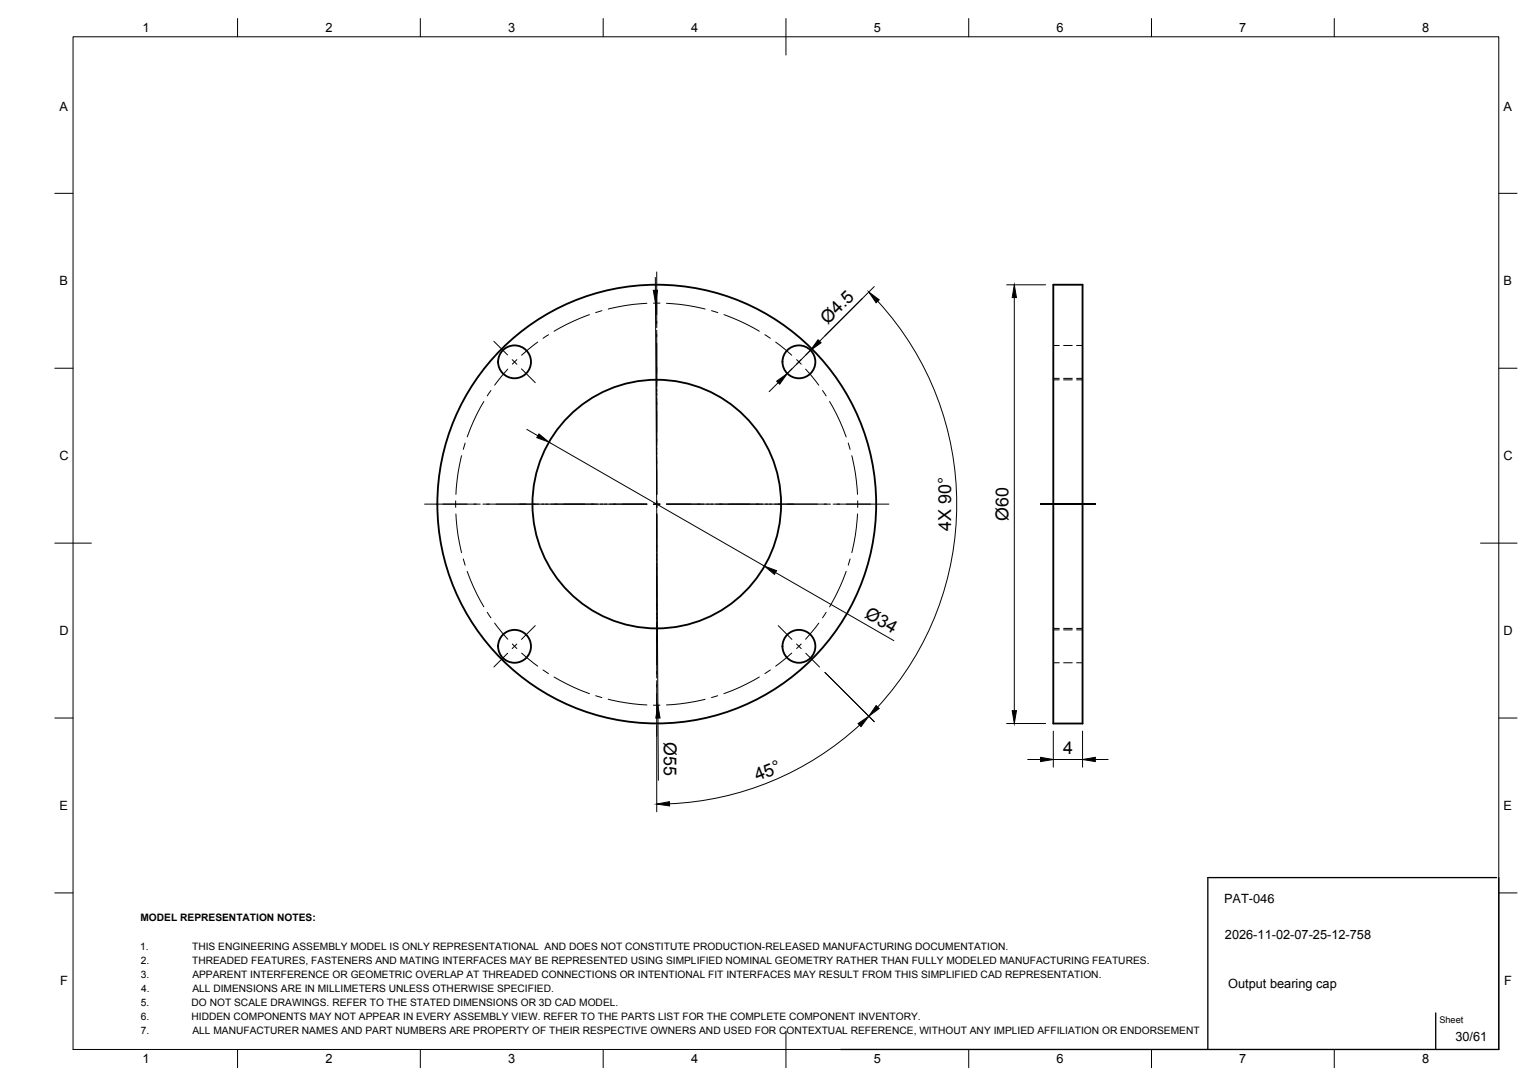
ISO-10303-21;
HEADER;
/* Generated by software containing ST-Developer
 * from STEP Tools, Inc. (www.steptools.com) 
 */

FILE_DESCRIPTION(
/* description */ ('Gear mesh backlash fixture'),
/* implementation_level */ '2;1');

FILE_NAME(
/* name */ 'Output bearing cap.step',
/* time_stamp */ '2026-10-28T03:26:00-07:00',
/* author */ (''),
/* organization */ (''),
/* preprocessor_version */ 'ST-DEVELOPER v20.2',
/* originating_system */ 'Autodesk Translation Framework v15.17.0.0',
/* authorisation */ '');

FILE_SCHEMA (('AUTOMOTIVE_DESIGN { 1 0 10303 214 3 1 1 }'));
ENDSEC;

DATA;
#10=MECHANICAL_DESIGN_GEOMETRIC_PRESENTATION_REPRESENTATION('',(#1045),#57900);
#938=SHAPE_REPRESENTATION_RELATIONSHIP('SRR','None',#58135,#988);
#988=ADVANCED_BREP_SHAPE_REPRESENTATION('',(#1109),#57868);
#1045=STYLED_ITEM('',(#58465),#1109);
#1109=MANIFOLD_SOLID_BREP('Body1',#13606);
#1266=FACE_BOUND('',#2861,.T.);
#1267=FACE_BOUND('',#2862,.T.);
#1268=FACE_BOUND('',#2863,.T.);
#1269=FACE_BOUND('',#2864,.T.);
#1270=FACE_BOUND('',#2865,.T.);
#1271=FACE_BOUND('',#2867,.T.);
#1272=FACE_BOUND('',#2868,.T.);
#1273=FACE_BOUND('',#2869,.T.);
#1274=FACE_BOUND('',#2870,.T.);
#1275=FACE_BOUND('',#2871,.T.);
#1472=PLANE('',#14799);
#1473=PLANE('',#14800);
#1966=FACE_OUTER_BOUND('',#2854,.T.);
#1967=FACE_OUTER_BOUND('',#2855,.T.);
#1968=FACE_OUTER_BOUND('',#2856,.T.);
#1969=FACE_OUTER_BOUND('',#2857,.T.);
#1970=FACE_OUTER_BOUND('',#2858,.T.);
#1971=FACE_OUTER_BOUND('',#2859,.T.);
#1972=FACE_OUTER_BOUND('',#2860,.T.);
#1973=FACE_OUTER_BOUND('',#2866,.T.);
#2854=EDGE_LOOP('',(#10089,#10090,#10091,#10092));
#2855=EDGE_LOOP('',(#10093,#10094,#10095,#10096));
#2856=EDGE_LOOP('',(#10097,#10098,#10099,#10100));
#2857=EDGE_LOOP('',(#10101,#10102,#10103,#10104));
#2858=EDGE_LOOP('',(#10105,#10106,#10107,#10108));
#2859=EDGE_LOOP('',(#10109,#10110,#10111,#10112));
#2860=EDGE_LOOP('',(#10113));
#2861=EDGE_LOOP('',(#10114));
#2862=EDGE_LOOP('',(#10115));
#2863=EDGE_LOOP('',(#10116));
#2864=EDGE_LOOP('',(#10117));
#2865=EDGE_LOOP('',(#10118));
#2866=EDGE_LOOP('',(#10119));
#2867=EDGE_LOOP('',(#10120));
#2868=EDGE_LOOP('',(#10121));
#2869=EDGE_LOOP('',(#10122));
#2870=EDGE_LOOP('',(#10123));
#2871=EDGE_LOOP('',(#10124));
#3709=LINE('',#21009,#4598);
#3710=LINE('',#21015,#4599);
#3711=LINE('',#21021,#4600);
#3712=LINE('',#21027,#4601);
#3713=LINE('',#21033,#4602);
#3714=LINE('',#21039,#4603);
#4598=VECTOR('',#17052,0.225);
#4599=VECTOR('',#17059,0.225);
#4600=VECTOR('',#17066,0.225);
#4601=VECTOR('',#17073,0.225000000000001);
#4602=VECTOR('',#17080,1.7);
#4603=VECTOR('',#17087,3.);
#5471=CIRCLE('',#14782,0.225);
#5472=CIRCLE('',#14783,0.225);
#5473=CIRCLE('',#14785,0.225);
#5474=CIRCLE('',#14786,0.225);
#5475=CIRCLE('',#14788,0.225);
#5476=CIRCLE('',#14789,0.225);
#5477=CIRCLE('',#14791,0.225000000000001);
#5478=CIRCLE('',#14792,0.225000000000001);
#5479=CIRCLE('',#14794,1.7);
#5480=CIRCLE('',#14795,1.7);
#5481=CIRCLE('',#14797,3.);
#5482=CIRCLE('',#14798,3.);
#6187=VERTEX_POINT('',#21006);
#6188=VERTEX_POINT('',#21008);
#6189=VERTEX_POINT('',#21012);
#6190=VERTEX_POINT('',#21014);
#6191=VERTEX_POINT('',#21018);
#6192=VERTEX_POINT('',#21020);
#6193=VERTEX_POINT('',#21024);
#6194=VERTEX_POINT('',#21026);
#6195=VERTEX_POINT('',#21030);
#6196=VERTEX_POINT('',#21032);
#6197=VERTEX_POINT('',#21036);
#6198=VERTEX_POINT('',#21038);
#7631=EDGE_CURVE('',#6187,#6187,#5471,.T.);
#7632=EDGE_CURVE('',#6187,#6188,#3709,.T.);
#7633=EDGE_CURVE('',#6188,#6188,#5472,.T.);
#7634=EDGE_CURVE('',#6189,#6189,#5473,.T.);
#7635=EDGE_CURVE('',#6189,#6190,#3710,.T.);
#7636=EDGE_CURVE('',#6190,#6190,#5474,.T.);
#7637=EDGE_CURVE('',#6191,#6191,#5475,.T.);
#7638=EDGE_CURVE('',#6191,#6192,#3711,.T.);
#7639=EDGE_CURVE('',#6192,#6192,#5476,.T.);
#7640=EDGE_CURVE('',#6193,#6193,#5477,.T.);
#7641=EDGE_CURVE('',#6193,#6194,#3712,.T.);
#7642=EDGE_CURVE('',#6194,#6194,#5478,.T.);
#7643=EDGE_CURVE('',#6195,#6195,#5479,.T.);
#7644=EDGE_CURVE('',#6195,#6196,#3713,.T.);
#7645=EDGE_CURVE('',#6196,#6196,#5480,.T.);
#7646=EDGE_CURVE('',#6197,#6197,#5481,.T.);
#7647=EDGE_CURVE('',#6197,#6198,#3714,.T.);
#7648=EDGE_CURVE('',#6198,#6198,#5482,.T.);
#10089=ORIENTED_EDGE('',*,*,#7631,.F.);
#10090=ORIENTED_EDGE('',*,*,#7632,.T.);
#10091=ORIENTED_EDGE('',*,*,#7633,.F.);
#10092=ORIENTED_EDGE('',*,*,#7632,.F.);
#10093=ORIENTED_EDGE('',*,*,#7634,.F.);
#10094=ORIENTED_EDGE('',*,*,#7635,.T.);
#10095=ORIENTED_EDGE('',*,*,#7636,.F.);
#10096=ORIENTED_EDGE('',*,*,#7635,.F.);
#10097=ORIENTED_EDGE('',*,*,#7637,.F.);
#10098=ORIENTED_EDGE('',*,*,#7638,.T.);
#10099=ORIENTED_EDGE('',*,*,#7639,.F.);
#10100=ORIENTED_EDGE('',*,*,#7638,.F.);
#10101=ORIENTED_EDGE('',*,*,#7640,.F.);
#10102=ORIENTED_EDGE('',*,*,#7641,.T.);
#10103=ORIENTED_EDGE('',*,*,#7642,.F.);
#10104=ORIENTED_EDGE('',*,*,#7641,.F.);
#10105=ORIENTED_EDGE('',*,*,#7643,.F.);
#10106=ORIENTED_EDGE('',*,*,#7644,.T.);
#10107=ORIENTED_EDGE('',*,*,#7645,.T.);
#10108=ORIENTED_EDGE('',*,*,#7644,.F.);
#10109=ORIENTED_EDGE('',*,*,#7646,.F.);
#10110=ORIENTED_EDGE('',*,*,#7647,.T.);
#10111=ORIENTED_EDGE('',*,*,#7648,.T.);
#10112=ORIENTED_EDGE('',*,*,#7647,.F.);
#10113=ORIENTED_EDGE('',*,*,#7646,.T.);
#10114=ORIENTED_EDGE('',*,*,#7643,.T.);
#10115=ORIENTED_EDGE('',*,*,#7642,.T.);
#10116=ORIENTED_EDGE('',*,*,#7639,.T.);
#10117=ORIENTED_EDGE('',*,*,#7636,.T.);
#10118=ORIENTED_EDGE('',*,*,#7633,.T.);
#10119=ORIENTED_EDGE('',*,*,#7648,.F.);
#10120=ORIENTED_EDGE('',*,*,#7645,.F.);
#10121=ORIENTED_EDGE('',*,*,#7640,.T.);
#10122=ORIENTED_EDGE('',*,*,#7637,.T.);
#10123=ORIENTED_EDGE('',*,*,#7634,.T.);
#10124=ORIENTED_EDGE('',*,*,#7631,.T.);
#12691=CYLINDRICAL_SURFACE('',#14781,0.225);
#12692=CYLINDRICAL_SURFACE('',#14784,0.225);
#12693=CYLINDRICAL_SURFACE('',#14787,0.225);
#12694=CYLINDRICAL_SURFACE('',#14790,0.225000000000001);
#12695=CYLINDRICAL_SURFACE('',#14793,1.7);
#12696=CYLINDRICAL_SURFACE('',#14796,3.);
#13083=ADVANCED_FACE('',(#1966),#12691,.F.);
#13084=ADVANCED_FACE('',(#1967),#12692,.F.);
#13085=ADVANCED_FACE('',(#1968),#12693,.F.);
#13086=ADVANCED_FACE('',(#1969),#12694,.F.);
#13087=ADVANCED_FACE('',(#1970),#12695,.F.);
#13088=ADVANCED_FACE('',(#1971),#12696,.T.);
#13089=ADVANCED_FACE('',(#1972,#1266,#1267,#1268,#1269,#1270),#1472,.T.);
#13090=ADVANCED_FACE('',(#1973,#1271,#1272,#1273,#1274,#1275),#1473,.F.);
#13606=CLOSED_SHELL('',(#13083,#13084,#13085,#13086,#13087,#13088,#13089,
#13090));
#14780=AXIS2_PLACEMENT_3D('',#21004,#17046,#17047);
#14781=AXIS2_PLACEMENT_3D('',#21005,#17048,#17049);
#14782=AXIS2_PLACEMENT_3D('',#21007,#17050,#17051);
#14783=AXIS2_PLACEMENT_3D('',#21010,#17053,#17054);
#14784=AXIS2_PLACEMENT_3D('',#21011,#17055,#17056);
#14785=AXIS2_PLACEMENT_3D('',#21013,#17057,#17058);
#14786=AXIS2_PLACEMENT_3D('',#21016,#17060,#17061);
#14787=AXIS2_PLACEMENT_3D('',#21017,#17062,#17063);
#14788=AXIS2_PLACEMENT_3D('',#21019,#17064,#17065);
#14789=AXIS2_PLACEMENT_3D('',#21022,#17067,#17068);
#14790=AXIS2_PLACEMENT_3D('',#21023,#17069,#17070);
#14791=AXIS2_PLACEMENT_3D('',#21025,#17071,#17072);
#14792=AXIS2_PLACEMENT_3D('',#21028,#17074,#17075);
#14793=AXIS2_PLACEMENT_3D('',#21029,#17076,#17077);
#14794=AXIS2_PLACEMENT_3D('',#21031,#17078,#17079);
#14795=AXIS2_PLACEMENT_3D('',#21034,#17081,#17082);
#14796=AXIS2_PLACEMENT_3D('',#21035,#17083,#17084);
#14797=AXIS2_PLACEMENT_3D('',#21037,#17085,#17086);
#14798=AXIS2_PLACEMENT_3D('',#21040,#17088,#17089);
#14799=AXIS2_PLACEMENT_3D('',#21041,#17090,#17091);
#14800=AXIS2_PLACEMENT_3D('',#21042,#17092,#17093);
#17046=DIRECTION('axis',(0.,0.,1.));
#17047=DIRECTION('refdir',(1.,0.,0.));
#17048=DIRECTION('center_axis',(0.,0.,1.));
#17049=DIRECTION('ref_axis',(1.,0.,0.));
#17050=DIRECTION('center_axis',(0.,0.,1.));
#17051=DIRECTION('ref_axis',(1.,0.,0.));
#17052=DIRECTION('',(0.,0.,1.));
#17053=DIRECTION('center_axis',(0.,0.,-1.));
#17054=DIRECTION('ref_axis',(1.,0.,0.));
#17055=DIRECTION('center_axis',(0.,0.,1.));
#17056=DIRECTION('ref_axis',(1.,0.,0.));
#17057=DIRECTION('center_axis',(0.,0.,1.));
#17058=DIRECTION('ref_axis',(1.,0.,0.));
#17059=DIRECTION('',(0.,0.,1.));
#17060=DIRECTION('center_axis',(0.,0.,-1.));
#17061=DIRECTION('ref_axis',(1.,0.,0.));
#17062=DIRECTION('center_axis',(0.,0.,1.));
#17063=DIRECTION('ref_axis',(1.,0.,0.));
#17064=DIRECTION('center_axis',(0.,0.,1.));
#17065=DIRECTION('ref_axis',(1.,0.,0.));
#17066=DIRECTION('',(0.,0.,1.));
#17067=DIRECTION('center_axis',(0.,0.,-1.));
#17068=DIRECTION('ref_axis',(1.,0.,0.));
#17069=DIRECTION('center_axis',(0.,0.,1.));
#17070=DIRECTION('ref_axis',(1.,0.,0.));
#17071=DIRECTION('center_axis',(0.,0.,1.));
#17072=DIRECTION('ref_axis',(1.,0.,0.));
#17073=DIRECTION('',(0.,0.,1.));
#17074=DIRECTION('center_axis',(0.,0.,-1.));
#17075=DIRECTION('ref_axis',(1.,0.,0.));
#17076=DIRECTION('center_axis',(0.,0.,1.));
#17077=DIRECTION('ref_axis',(1.,0.,0.));
#17078=DIRECTION('center_axis',(0.,0.,-1.));
#17079=DIRECTION('ref_axis',(1.,0.,0.));
#17080=DIRECTION('',(0.,0.,-1.));
#17081=DIRECTION('center_axis',(0.,0.,-1.));
#17082=DIRECTION('ref_axis',(1.,0.,0.));
#17083=DIRECTION('center_axis',(0.,0.,1.));
#17084=DIRECTION('ref_axis',(1.,0.,0.));
#17085=DIRECTION('center_axis',(0.,0.,1.));
#17086=DIRECTION('ref_axis',(1.,0.,0.));
#17087=DIRECTION('',(0.,0.,-1.));
#17088=DIRECTION('center_axis',(0.,0.,1.));
#17089=DIRECTION('ref_axis',(1.,0.,0.));
#17090=DIRECTION('center_axis',(0.,0.,1.));
#17091=DIRECTION('ref_axis',(1.,0.,0.));
#17092=DIRECTION('center_axis',(0.,0.,1.));
#17093=DIRECTION('ref_axis',(1.,0.,0.));
#21004=CARTESIAN_POINT('',(0.,0.,0.));
#21005=CARTESIAN_POINT('Origin',(4.05545635173699,-1.94454364826301,9.1));
#21006=CARTESIAN_POINT('',(3.83045635173699,-1.94454364826301,9.2));
#21007=CARTESIAN_POINT('Origin',(4.05545635173699,-1.94454364826301,9.2));
#21008=CARTESIAN_POINT('',(3.83045635173699,-1.94454364826301,9.6));
#21009=CARTESIAN_POINT('',(3.83045635173699,-1.94454364826301,9.1));
#21010=CARTESIAN_POINT('Origin',(4.05545635173699,-1.94454364826301,9.6));
#21011=CARTESIAN_POINT('Origin',(4.05545635173699,1.94454364826301,9.1));
#21012=CARTESIAN_POINT('',(3.83045635173699,1.94454364826301,9.2));
#21013=CARTESIAN_POINT('Origin',(4.05545635173699,1.94454364826301,9.2));
#21014=CARTESIAN_POINT('',(3.83045635173699,1.94454364826301,9.6));
#21015=CARTESIAN_POINT('',(3.83045635173699,1.94454364826301,9.1));
#21016=CARTESIAN_POINT('Origin',(4.05545635173699,1.94454364826301,9.6));
#21017=CARTESIAN_POINT('Origin',(7.94454364826301,1.94454364826301,9.1));
#21018=CARTESIAN_POINT('',(7.71954364826301,1.94454364826301,9.2));
#21019=CARTESIAN_POINT('Origin',(7.94454364826301,1.94454364826301,9.2));
#21020=CARTESIAN_POINT('',(7.71954364826301,1.94454364826301,9.6));
#21021=CARTESIAN_POINT('',(7.71954364826301,1.94454364826301,9.1));
#21022=CARTESIAN_POINT('Origin',(7.94454364826301,1.94454364826301,9.6));
#21023=CARTESIAN_POINT('Origin',(7.944543648263,-1.94454364826301,9.1));
#21024=CARTESIAN_POINT('',(7.719543648263,-1.94454364826301,9.2));
#21025=CARTESIAN_POINT('Origin',(7.944543648263,-1.94454364826301,9.2));
#21026=CARTESIAN_POINT('',(7.719543648263,-1.94454364826301,9.6));
#21027=CARTESIAN_POINT('',(7.719543648263,-1.94454364826301,9.1));
#21028=CARTESIAN_POINT('Origin',(7.944543648263,-1.94454364826301,9.6));
#21029=CARTESIAN_POINT('Origin',(6.,0.,9.2));
#21030=CARTESIAN_POINT('',(4.3,-2.0818995585505E-16,9.6));
#21031=CARTESIAN_POINT('Origin',(6.,0.,9.6));
#21032=CARTESIAN_POINT('',(4.3,-2.0818995585505E-16,9.2));
#21033=CARTESIAN_POINT('',(4.3,-2.0818995585505E-16,9.2));
#21034=CARTESIAN_POINT('Origin',(6.,0.,9.2));
#21035=CARTESIAN_POINT('Origin',(6.,0.,9.2));
#21036=CARTESIAN_POINT('',(3.,-3.67394039744206E-16,9.6));
#21037=CARTESIAN_POINT('Origin',(6.,0.,9.6));
#21038=CARTESIAN_POINT('',(3.,-3.67394039744206E-16,9.2));
#21039=CARTESIAN_POINT('',(3.,-3.67394039744206E-16,9.2));
#21040=CARTESIAN_POINT('Origin',(6.,0.,9.2));
#21041=CARTESIAN_POINT('Origin',(6.,0.,9.6));
#21042=CARTESIAN_POINT('Origin',(6.,0.,9.2));
#57809=UNCERTAINTY_MEASURE_WITH_UNIT(LENGTH_MEASURE(0.001),#57901,
'DISTANCE_ACCURACY_VALUE',
'Maximum model space distance between geometric entities at asserted c
onnectivities');
#57841=UNCERTAINTY_MEASURE_WITH_UNIT(LENGTH_MEASURE(0.001),#57901,
'DISTANCE_ACCURACY_VALUE',
'Maximum model space distance between geometric entities at asserted c
onnectivities');
#57868=(
GEOMETRIC_REPRESENTATION_CONTEXT(3)
GLOBAL_UNCERTAINTY_ASSIGNED_CONTEXT((#57809))
GLOBAL_UNIT_ASSIGNED_CONTEXT((#57901,#57903,#57904))
REPRESENTATION_CONTEXT('','3D')
);
#57900=(
GEOMETRIC_REPRESENTATION_CONTEXT(3)
GLOBAL_UNCERTAINTY_ASSIGNED_CONTEXT((#57841))
GLOBAL_UNIT_ASSIGNED_CONTEXT((#57901,#57903,#57904))
REPRESENTATION_CONTEXT('','3D')
);
#57901=(
LENGTH_UNIT()
NAMED_UNIT(*)
SI_UNIT(.CENTI.,.METRE.)
);
#57903=(
NAMED_UNIT(*)
PLANE_ANGLE_UNIT()
SI_UNIT($,.RADIAN.)
);
#57904=(
NAMED_UNIT(*)
SI_UNIT($,.STERADIAN.)
SOLID_ANGLE_UNIT()
);
#57931=SHAPE_DEFINITION_REPRESENTATION(#57994,#58135);
#57994=PRODUCT_DEFINITION_SHAPE('',$,#58194);
#58135=SHAPE_REPRESENTATION('',(#14780),#57868);
#58167=PRODUCT_DEFINITION_CONTEXT('part definition',#58343,'design');
#58194=PRODUCT_DEFINITION('Output bearing cap','Output bearing cap',#58252,
#58167);
#58252=PRODUCT_DEFINITION_FORMATION('',$,#58371);
#58343=APPLICATION_CONTEXT(
'Core Data for Automotive Mechanical Design Process');
#58344=PRODUCT_CONTEXT('part definition',#58343,'mechanical');
#58371=PRODUCT('Output bearing cap','Output bearing cap',
'Output bearing cap',(#58344));
#58459=COLOUR_RGB('Grey',0.48,0.52,0.57);
#58460=FILL_AREA_STYLE_COLOUR('',#58459);
#58461=FILL_AREA_STYLE('',(#58460));
#58462=SURFACE_STYLE_FILL_AREA(#58461);
#58463=SURFACE_SIDE_STYLE('',(#58462));
#58464=SURFACE_STYLE_USAGE(.BOTH.,#58463);
#58465=PRESENTATION_STYLE_ASSIGNMENT((#58464));
ENDSEC;
END-ISO-10303-21;
